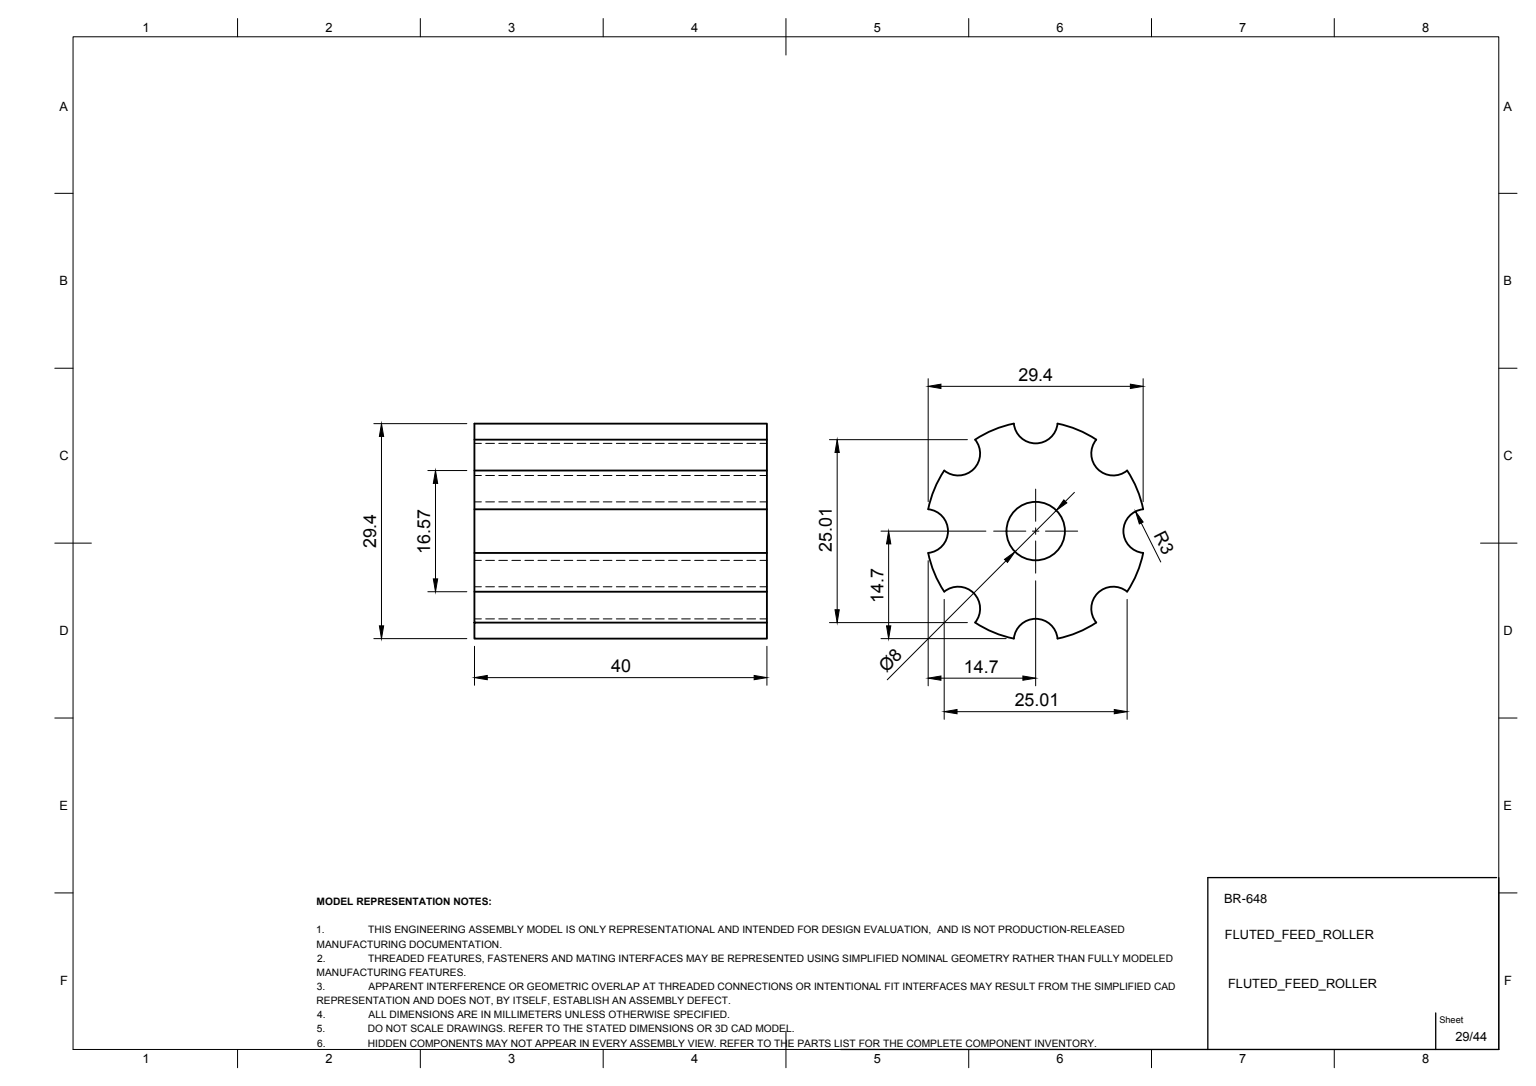
ISO-10303-21;
HEADER;
FILE_DESCRIPTION((''),'2;1');
FILE_NAME('FLUTED_FEED_ROLLER.step','2026-10-01T22:05:39-07:00',(''),(''),'','','');
FILE_SCHEMA (('AUTOMOTIVE_DESIGN { 1 0 10303 214 3 1 1 }'));
ENDSEC;
DATA;
#10=MECHANICAL_DESIGN_GEOMETRIC_PRESENTATION_REPRESENTATION('',(#627),#24628);
#543=SHAPE_REPRESENTATION_RELATIONSHIP('SRR','None',#24816,#585) ;
#585=ADVANCED_BREP_SHAPE_REPRESENTATION('',(#666),#24606) ;
#627=STYLED_ITEM('',(#25036),#666) ;
#666=MANIFOLD_SOLID_BREP('FLUTED_FEED_ROLLER',#13169) ;
#884=FACE_BOUND('',#4472,.T.) ;
#885=FACE_BOUND('',#4488,.T.) ;
#1542=LINE('',#23181,#2378) ;
#1543=LINE('',#23188,#2379) ;
#1544=LINE('',#23191,#2380) ;
#1545=LINE('',#23225,#2381) ;
#1546=LINE('',#23229,#2382) ;
#1547=LINE('',#23233,#2383) ;
#1548=LINE('',#23237,#2384) ;
#1549=LINE('',#23241,#2385) ;
#1550=LINE('',#23245,#2386) ;
#1551=LINE('',#23249,#2387) ;
#1552=LINE('',#23253,#2388) ;
#1553=LINE('',#23257,#2389) ;
#1554=LINE('',#23261,#2390) ;
#1555=LINE('',#23265,#2391) ;
#1556=LINE('',#23269,#2392) ;
#1557=LINE('',#23273,#2393) ;
#1558=LINE('',#23277,#2394) ;
#2378=VECTOR('',#18511,0.4) ;
#2379=VECTOR('',#18518,1.) ;
#2380=VECTOR('',#18521,1.) ;
#2381=VECTOR('',#18558,1.) ;
#2382=VECTOR('',#18563,1.) ;
#2383=VECTOR('',#18568,1.) ;
#2384=VECTOR('',#18573,1.) ;
#2385=VECTOR('',#18578,1.) ;
#2386=VECTOR('',#18583,1.) ;
#2387=VECTOR('',#18588,1.) ;
#2388=VECTOR('',#18593,1.) ;
#2389=VECTOR('',#18598,1.) ;
#2390=VECTOR('',#18603,1.) ;
#2391=VECTOR('',#18608,1.) ;
#2392=VECTOR('',#18613,1.) ;
#2393=VECTOR('',#18618,1.) ;
#2394=VECTOR('',#18623,1.) ;
#2880=CYLINDRICAL_SURFACE('',#14940,0.4) ;
#2881=CYLINDRICAL_SURFACE('',#14943,0.3) ;
#2882=CYLINDRICAL_SURFACE('',#14962,1.5) ;
#2883=CYLINDRICAL_SURFACE('',#14964,0.3) ;
#2884=CYLINDRICAL_SURFACE('',#14966,1.5) ;
#2885=CYLINDRICAL_SURFACE('',#14968,0.3) ;
#2886=CYLINDRICAL_SURFACE('',#14970,1.5) ;
#2887=CYLINDRICAL_SURFACE('',#14972,0.3) ;
#2888=CYLINDRICAL_SURFACE('',#14974,1.5) ;
#2889=CYLINDRICAL_SURFACE('',#14976,0.3) ;
#2890=CYLINDRICAL_SURFACE('',#14978,1.5) ;
#2891=CYLINDRICAL_SURFACE('',#14980,0.3) ;
#2892=CYLINDRICAL_SURFACE('',#14982,1.5) ;
#2893=CYLINDRICAL_SURFACE('',#14984,0.3) ;
#2894=CYLINDRICAL_SURFACE('',#14986,1.5) ;
#2895=CYLINDRICAL_SURFACE('',#14988,0.3) ;
#2896=CYLINDRICAL_SURFACE('',#14992,1.5) ;
#3504=FACE_OUTER_BOUND('',#4469,.T.) ;
#3505=FACE_OUTER_BOUND('',#4470,.T.) ;
#3506=FACE_OUTER_BOUND('',#4471,.T.) ;
#3507=FACE_OUTER_BOUND('',#4473,.T.) ;
#3508=FACE_OUTER_BOUND('',#4474,.T.) ;
#3509=FACE_OUTER_BOUND('',#4475,.T.) ;
#3510=FACE_OUTER_BOUND('',#4476,.T.) ;
#3511=FACE_OUTER_BOUND('',#4477,.T.) ;
#3512=FACE_OUTER_BOUND('',#4478,.T.) ;
#3513=FACE_OUTER_BOUND('',#4479,.T.) ;
#3514=FACE_OUTER_BOUND('',#4480,.T.) ;
#3515=FACE_OUTER_BOUND('',#4481,.T.) ;
#3516=FACE_OUTER_BOUND('',#4482,.T.) ;
#3517=FACE_OUTER_BOUND('',#4483,.T.) ;
#3518=FACE_OUTER_BOUND('',#4484,.T.) ;
#3519=FACE_OUTER_BOUND('',#4485,.T.) ;
#3520=FACE_OUTER_BOUND('',#4486,.T.) ;
#3521=FACE_OUTER_BOUND('',#4487,.T.) ;
#3522=FACE_OUTER_BOUND('',#4489,.T.) ;
#4469=EDGE_LOOP('',(#11027,#11028,#11029,#11030)) ;
#4470=EDGE_LOOP('',(#11031,#11032,#11033,#11034)) ;
#4471=EDGE_LOOP('',(#11035,#11036,#11037,#11038,#11039,#11040,#11041,#11042,
#11043,#11044,#11045,#11046,#11047,#11048,#11049,#11050)) ;
#4472=EDGE_LOOP('',(#11051)) ;
#4473=EDGE_LOOP('',(#11052,#11053,#11054,#11055)) ;
#4474=EDGE_LOOP('',(#11056,#11057,#11058,#11059)) ;
#4475=EDGE_LOOP('',(#11060,#11061,#11062,#11063)) ;
#4476=EDGE_LOOP('',(#11064,#11065,#11066,#11067)) ;
#4477=EDGE_LOOP('',(#11068,#11069,#11070,#11071)) ;
#4478=EDGE_LOOP('',(#11072,#11073,#11074,#11075)) ;
#4479=EDGE_LOOP('',(#11076,#11077,#11078,#11079)) ;
#4480=EDGE_LOOP('',(#11080,#11081,#11082,#11083)) ;
#4481=EDGE_LOOP('',(#11084,#11085,#11086,#11087)) ;
#4482=EDGE_LOOP('',(#11088,#11089,#11090,#11091)) ;
#4483=EDGE_LOOP('',(#11092,#11093,#11094,#11095)) ;
#4484=EDGE_LOOP('',(#11096,#11097,#11098,#11099)) ;
#4485=EDGE_LOOP('',(#11100,#11101,#11102,#11103)) ;
#4486=EDGE_LOOP('',(#11104,#11105,#11106,#11107)) ;
#4487=EDGE_LOOP('',(#11108,#11109,#11110,#11111,#11112,#11113,#11114,#11115,
#11116,#11117,#11118,#11119,#11120,#11121,#11122,#11123)) ;
#4488=EDGE_LOOP('',(#11124)) ;
#4489=EDGE_LOOP('',(#11125,#11126,#11127,#11128)) ;
#5371=CIRCLE('',#14941,0.4) ;
#5372=CIRCLE('',#14942,0.4) ;
#5373=CIRCLE('',#14944,0.3) ;
#5374=CIRCLE('',#14945,0.3) ;
#5375=CIRCLE('',#14947,1.5) ;
#5376=CIRCLE('',#14948,0.3) ;
#5377=CIRCLE('',#14949,1.5) ;
#5378=CIRCLE('',#14950,0.3) ;
#5379=CIRCLE('',#14951,1.5) ;
#5380=CIRCLE('',#14952,0.3) ;
#5381=CIRCLE('',#14953,1.5) ;
#5382=CIRCLE('',#14954,0.3) ;
#5383=CIRCLE('',#14955,1.5) ;
#5384=CIRCLE('',#14956,0.3) ;
#5385=CIRCLE('',#14957,1.5) ;
#5386=CIRCLE('',#14958,0.3) ;
#5387=CIRCLE('',#14959,1.5) ;
#5388=CIRCLE('',#14960,0.3) ;
#5389=CIRCLE('',#14961,1.5) ;
#5390=CIRCLE('',#14963,1.5) ;
#5391=CIRCLE('',#14965,0.3) ;
#5392=CIRCLE('',#14967,1.5) ;
#5393=CIRCLE('',#14969,0.3) ;
#5394=CIRCLE('',#14971,1.5) ;
#5395=CIRCLE('',#14973,0.3) ;
#5396=CIRCLE('',#14975,1.5) ;
#5397=CIRCLE('',#14977,0.3) ;
#5398=CIRCLE('',#14979,1.5) ;
#5399=CIRCLE('',#14981,0.3) ;
#5400=CIRCLE('',#14983,1.5) ;
#5401=CIRCLE('',#14985,0.3) ;
#5402=CIRCLE('',#14987,1.5) ;
#5403=CIRCLE('',#14989,0.3) ;
#5404=CIRCLE('',#14991,1.5) ;
#6413=VERTEX_POINT('',#23178) ;
#6414=VERTEX_POINT('',#23180) ;
#6415=VERTEX_POINT('',#23184) ;
#6416=VERTEX_POINT('',#23185) ;
#6417=VERTEX_POINT('',#23187) ;
#6418=VERTEX_POINT('',#23189) ;
#6419=VERTEX_POINT('',#23193) ;
#6420=VERTEX_POINT('',#23195) ;
#6421=VERTEX_POINT('',#23197) ;
#6422=VERTEX_POINT('',#23199) ;
#6423=VERTEX_POINT('',#23201) ;
#6424=VERTEX_POINT('',#23203) ;
#6425=VERTEX_POINT('',#23205) ;
#6426=VERTEX_POINT('',#23207) ;
#6427=VERTEX_POINT('',#23209) ;
#6428=VERTEX_POINT('',#23211) ;
#6429=VERTEX_POINT('',#23213) ;
#6430=VERTEX_POINT('',#23215) ;
#6431=VERTEX_POINT('',#23217) ;
#6432=VERTEX_POINT('',#23219) ;
#6433=VERTEX_POINT('',#23223) ;
#6434=VERTEX_POINT('',#23227) ;
#6435=VERTEX_POINT('',#23231) ;
#6436=VERTEX_POINT('',#23235) ;
#6437=VERTEX_POINT('',#23239) ;
#6438=VERTEX_POINT('',#23243) ;
#6439=VERTEX_POINT('',#23247) ;
#6440=VERTEX_POINT('',#23251) ;
#6441=VERTEX_POINT('',#23255) ;
#6442=VERTEX_POINT('',#23259) ;
#6443=VERTEX_POINT('',#23263) ;
#6444=VERTEX_POINT('',#23267) ;
#6445=VERTEX_POINT('',#23271) ;
#6446=VERTEX_POINT('',#23275) ;
#8003=EDGE_CURVE('',#6413,#6413,#5371,.T.) ;
#8004=EDGE_CURVE('',#6413,#6414,#1542,.T.) ;
#8005=EDGE_CURVE('',#6414,#6414,#5372,.T.) ;
#8006=EDGE_CURVE('',#6415,#6416,#5373,.T.) ;
#8007=EDGE_CURVE('',#6417,#6415,#1543,.T.) ;
#8008=EDGE_CURVE('',#6418,#6417,#5374,.T.) ;
#8009=EDGE_CURVE('',#6416,#6418,#1544,.T.) ;
#8010=EDGE_CURVE('',#6417,#6419,#5375,.T.) ;
#8011=EDGE_CURVE('',#6419,#6420,#5376,.T.) ;
#8012=EDGE_CURVE('',#6420,#6421,#5377,.T.) ;
#8013=EDGE_CURVE('',#6421,#6422,#5378,.T.) ;
#8014=EDGE_CURVE('',#6422,#6423,#5379,.T.) ;
#8015=EDGE_CURVE('',#6423,#6424,#5380,.T.) ;
#8016=EDGE_CURVE('',#6424,#6425,#5381,.T.) ;
#8017=EDGE_CURVE('',#6425,#6426,#5382,.T.) ;
#8018=EDGE_CURVE('',#6426,#6427,#5383,.T.) ;
#8019=EDGE_CURVE('',#6427,#6428,#5384,.T.) ;
#8020=EDGE_CURVE('',#6428,#6429,#5385,.T.) ;
#8021=EDGE_CURVE('',#6429,#6430,#5386,.T.) ;
#8022=EDGE_CURVE('',#6430,#6431,#5387,.T.) ;
#8023=EDGE_CURVE('',#6431,#6432,#5388,.T.) ;
#8024=EDGE_CURVE('',#6432,#6418,#5389,.T.) ;
#8025=EDGE_CURVE('',#6433,#6415,#5390,.T.) ;
#8026=EDGE_CURVE('',#6433,#6419,#1545,.T.) ;
#8027=EDGE_CURVE('',#6434,#6433,#5391,.T.) ;
#8028=EDGE_CURVE('',#6420,#6434,#1546,.T.) ;
#8029=EDGE_CURVE('',#6435,#6434,#5392,.T.) ;
#8030=EDGE_CURVE('',#6435,#6421,#1547,.T.) ;
#8031=EDGE_CURVE('',#6436,#6435,#5393,.T.) ;
#8032=EDGE_CURVE('',#6422,#6436,#1548,.T.) ;
#8033=EDGE_CURVE('',#6437,#6436,#5394,.T.) ;
#8034=EDGE_CURVE('',#6437,#6423,#1549,.T.) ;
#8035=EDGE_CURVE('',#6438,#6437,#5395,.T.) ;
#8036=EDGE_CURVE('',#6424,#6438,#1550,.T.) ;
#8037=EDGE_CURVE('',#6439,#6438,#5396,.T.) ;
#8038=EDGE_CURVE('',#6439,#6425,#1551,.T.) ;
#8039=EDGE_CURVE('',#6440,#6439,#5397,.T.) ;
#8040=EDGE_CURVE('',#6426,#6440,#1552,.T.) ;
#8041=EDGE_CURVE('',#6441,#6440,#5398,.T.) ;
#8042=EDGE_CURVE('',#6441,#6427,#1553,.T.) ;
#8043=EDGE_CURVE('',#6442,#6441,#5399,.T.) ;
#8044=EDGE_CURVE('',#6428,#6442,#1554,.T.) ;
#8045=EDGE_CURVE('',#6443,#6442,#5400,.T.) ;
#8046=EDGE_CURVE('',#6443,#6429,#1555,.T.) ;
#8047=EDGE_CURVE('',#6444,#6443,#5401,.T.) ;
#8048=EDGE_CURVE('',#6430,#6444,#1556,.T.) ;
#8049=EDGE_CURVE('',#6445,#6444,#5402,.T.) ;
#8050=EDGE_CURVE('',#6445,#6431,#1557,.T.) ;
#8051=EDGE_CURVE('',#6446,#6445,#5403,.T.) ;
#8052=EDGE_CURVE('',#6432,#6446,#1558,.T.) ;
#8053=EDGE_CURVE('',#6416,#6446,#5404,.T.) ;
#11027=ORIENTED_EDGE('',*,*,#8003,.F.) ;
#11028=ORIENTED_EDGE('',*,*,#8004,.T.) ;
#11029=ORIENTED_EDGE('',*,*,#8005,.F.) ;
#11030=ORIENTED_EDGE('',*,*,#8004,.F.) ;
#11031=ORIENTED_EDGE('',*,*,#8006,.F.) ;
#11032=ORIENTED_EDGE('',*,*,#8007,.F.) ;
#11033=ORIENTED_EDGE('',*,*,#8008,.F.) ;
#11034=ORIENTED_EDGE('',*,*,#8009,.F.) ;
#11035=ORIENTED_EDGE('',*,*,#8008,.T.) ;
#11036=ORIENTED_EDGE('',*,*,#8010,.T.) ;
#11037=ORIENTED_EDGE('',*,*,#8011,.T.) ;
#11038=ORIENTED_EDGE('',*,*,#8012,.T.) ;
#11039=ORIENTED_EDGE('',*,*,#8013,.T.) ;
#11040=ORIENTED_EDGE('',*,*,#8014,.T.) ;
#11041=ORIENTED_EDGE('',*,*,#8015,.T.) ;
#11042=ORIENTED_EDGE('',*,*,#8016,.T.) ;
#11043=ORIENTED_EDGE('',*,*,#8017,.T.) ;
#11044=ORIENTED_EDGE('',*,*,#8018,.T.) ;
#11045=ORIENTED_EDGE('',*,*,#8019,.T.) ;
#11046=ORIENTED_EDGE('',*,*,#8020,.T.) ;
#11047=ORIENTED_EDGE('',*,*,#8021,.T.) ;
#11048=ORIENTED_EDGE('',*,*,#8022,.T.) ;
#11049=ORIENTED_EDGE('',*,*,#8023,.T.) ;
#11050=ORIENTED_EDGE('',*,*,#8024,.T.) ;
#11051=ORIENTED_EDGE('',*,*,#8005,.T.) ;
#11052=ORIENTED_EDGE('',*,*,#8007,.T.) ;
#11053=ORIENTED_EDGE('',*,*,#8025,.F.) ;
#11054=ORIENTED_EDGE('',*,*,#8026,.T.) ;
#11055=ORIENTED_EDGE('',*,*,#8010,.F.) ;
#11056=ORIENTED_EDGE('',*,*,#8027,.F.) ;
#11057=ORIENTED_EDGE('',*,*,#8028,.F.) ;
#11058=ORIENTED_EDGE('',*,*,#8011,.F.) ;
#11059=ORIENTED_EDGE('',*,*,#8026,.F.) ;
#11060=ORIENTED_EDGE('',*,*,#8028,.T.) ;
#11061=ORIENTED_EDGE('',*,*,#8029,.F.) ;
#11062=ORIENTED_EDGE('',*,*,#8030,.T.) ;
#11063=ORIENTED_EDGE('',*,*,#8012,.F.) ;
#11064=ORIENTED_EDGE('',*,*,#8031,.F.) ;
#11065=ORIENTED_EDGE('',*,*,#8032,.F.) ;
#11066=ORIENTED_EDGE('',*,*,#8013,.F.) ;
#11067=ORIENTED_EDGE('',*,*,#8030,.F.) ;
#11068=ORIENTED_EDGE('',*,*,#8032,.T.) ;
#11069=ORIENTED_EDGE('',*,*,#8033,.F.) ;
#11070=ORIENTED_EDGE('',*,*,#8034,.T.) ;
#11071=ORIENTED_EDGE('',*,*,#8014,.F.) ;
#11072=ORIENTED_EDGE('',*,*,#8035,.F.) ;
#11073=ORIENTED_EDGE('',*,*,#8036,.F.) ;
#11074=ORIENTED_EDGE('',*,*,#8015,.F.) ;
#11075=ORIENTED_EDGE('',*,*,#8034,.F.) ;
#11076=ORIENTED_EDGE('',*,*,#8036,.T.) ;
#11077=ORIENTED_EDGE('',*,*,#8037,.F.) ;
#11078=ORIENTED_EDGE('',*,*,#8038,.T.) ;
#11079=ORIENTED_EDGE('',*,*,#8016,.F.) ;
#11080=ORIENTED_EDGE('',*,*,#8039,.F.) ;
#11081=ORIENTED_EDGE('',*,*,#8040,.F.) ;
#11082=ORIENTED_EDGE('',*,*,#8017,.F.) ;
#11083=ORIENTED_EDGE('',*,*,#8038,.F.) ;
#11084=ORIENTED_EDGE('',*,*,#8040,.T.) ;
#11085=ORIENTED_EDGE('',*,*,#8041,.F.) ;
#11086=ORIENTED_EDGE('',*,*,#8042,.T.) ;
#11087=ORIENTED_EDGE('',*,*,#8018,.F.) ;
#11088=ORIENTED_EDGE('',*,*,#8043,.F.) ;
#11089=ORIENTED_EDGE('',*,*,#8044,.F.) ;
#11090=ORIENTED_EDGE('',*,*,#8019,.F.) ;
#11091=ORIENTED_EDGE('',*,*,#8042,.F.) ;
#11092=ORIENTED_EDGE('',*,*,#8044,.T.) ;
#11093=ORIENTED_EDGE('',*,*,#8045,.F.) ;
#11094=ORIENTED_EDGE('',*,*,#8046,.T.) ;
#11095=ORIENTED_EDGE('',*,*,#8020,.F.) ;
#11096=ORIENTED_EDGE('',*,*,#8047,.F.) ;
#11097=ORIENTED_EDGE('',*,*,#8048,.F.) ;
#11098=ORIENTED_EDGE('',*,*,#8021,.F.) ;
#11099=ORIENTED_EDGE('',*,*,#8046,.F.) ;
#11100=ORIENTED_EDGE('',*,*,#8048,.T.) ;
#11101=ORIENTED_EDGE('',*,*,#8049,.F.) ;
#11102=ORIENTED_EDGE('',*,*,#8050,.T.) ;
#11103=ORIENTED_EDGE('',*,*,#8022,.F.) ;
#11104=ORIENTED_EDGE('',*,*,#8050,.F.) ;
#11105=ORIENTED_EDGE('',*,*,#8051,.F.) ;
#11106=ORIENTED_EDGE('',*,*,#8052,.F.) ;
#11107=ORIENTED_EDGE('',*,*,#8023,.F.) ;
#11108=ORIENTED_EDGE('',*,*,#8006,.T.) ;
#11109=ORIENTED_EDGE('',*,*,#8053,.T.) ;
#11110=ORIENTED_EDGE('',*,*,#8051,.T.) ;
#11111=ORIENTED_EDGE('',*,*,#8049,.T.) ;
#11112=ORIENTED_EDGE('',*,*,#8047,.T.) ;
#11113=ORIENTED_EDGE('',*,*,#8045,.T.) ;
#11114=ORIENTED_EDGE('',*,*,#8043,.T.) ;
#11115=ORIENTED_EDGE('',*,*,#8041,.T.) ;
#11116=ORIENTED_EDGE('',*,*,#8039,.T.) ;
#11117=ORIENTED_EDGE('',*,*,#8037,.T.) ;
#11118=ORIENTED_EDGE('',*,*,#8035,.T.) ;
#11119=ORIENTED_EDGE('',*,*,#8033,.T.) ;
#11120=ORIENTED_EDGE('',*,*,#8031,.T.) ;
#11121=ORIENTED_EDGE('',*,*,#8029,.T.) ;
#11122=ORIENTED_EDGE('',*,*,#8027,.T.) ;
#11123=ORIENTED_EDGE('',*,*,#8025,.T.) ;
#11124=ORIENTED_EDGE('',*,*,#8003,.T.) ;
#11125=ORIENTED_EDGE('',*,*,#8009,.T.) ;
#11126=ORIENTED_EDGE('',*,*,#8024,.F.) ;
#11127=ORIENTED_EDGE('',*,*,#8052,.T.) ;
#11128=ORIENTED_EDGE('',*,*,#8053,.F.) ;
#12209=PLANE('',#14946) ;
#12210=PLANE('',#14990) ;
#12899=ADVANCED_FACE('',(#3504),#2880,.F.) ;
#12900=ADVANCED_FACE('',(#3505),#2881,.F.) ;
#12901=ADVANCED_FACE('',(#3506,#884),#12209,.T.) ;
#12902=ADVANCED_FACE('',(#3507),#2882,.T.) ;
#12903=ADVANCED_FACE('',(#3508),#2883,.F.) ;
#12904=ADVANCED_FACE('',(#3509),#2884,.T.) ;
#12905=ADVANCED_FACE('',(#3510),#2885,.F.) ;
#12906=ADVANCED_FACE('',(#3511),#2886,.T.) ;
#12907=ADVANCED_FACE('',(#3512),#2887,.F.) ;
#12908=ADVANCED_FACE('',(#3513),#2888,.T.) ;
#12909=ADVANCED_FACE('',(#3514),#2889,.F.) ;
#12910=ADVANCED_FACE('',(#3515),#2890,.T.) ;
#12911=ADVANCED_FACE('',(#3516),#2891,.F.) ;
#12912=ADVANCED_FACE('',(#3517),#2892,.T.) ;
#12913=ADVANCED_FACE('',(#3518),#2893,.F.) ;
#12914=ADVANCED_FACE('',(#3519),#2894,.T.) ;
#12915=ADVANCED_FACE('',(#3520),#2895,.F.) ;
#12916=ADVANCED_FACE('',(#3521,#885),#12210,.T.) ;
#12917=ADVANCED_FACE('',(#3522),#2896,.T.) ;
#13169=CLOSED_SHELL('',(#12899,#12900,#12901,#12902,#12903,#12904,#12905,
#12906,#12907,#12908,#12909,#12910,#12911,#12912,#12913,#12914,#12915,#12916,
#12917)) ;
#14939=AXIS2_PLACEMENT_3D('',#23176,#18505,#18506) ;
#14940=AXIS2_PLACEMENT_3D('',#23177,#18507,#18508) ;
#14941=AXIS2_PLACEMENT_3D('',#23179,#18509,#18510) ;
#14942=AXIS2_PLACEMENT_3D('',#23182,#18512,#18513) ;
#14943=AXIS2_PLACEMENT_3D('',#23183,#18514,#18515) ;
#14944=AXIS2_PLACEMENT_3D('',#23186,#18516,#18517) ;
#14945=AXIS2_PLACEMENT_3D('',#23190,#18519,#18520) ;
#14946=AXIS2_PLACEMENT_3D('',#23192,#18522,#18523) ;
#14947=AXIS2_PLACEMENT_3D('',#23194,#18524,#18525) ;
#14948=AXIS2_PLACEMENT_3D('',#23196,#18526,#18527) ;
#14949=AXIS2_PLACEMENT_3D('',#23198,#18528,#18529) ;
#14950=AXIS2_PLACEMENT_3D('',#23200,#18530,#18531) ;
#14951=AXIS2_PLACEMENT_3D('',#23202,#18532,#18533) ;
#14952=AXIS2_PLACEMENT_3D('',#23204,#18534,#18535) ;
#14953=AXIS2_PLACEMENT_3D('',#23206,#18536,#18537) ;
#14954=AXIS2_PLACEMENT_3D('',#23208,#18538,#18539) ;
#14955=AXIS2_PLACEMENT_3D('',#23210,#18540,#18541) ;
#14956=AXIS2_PLACEMENT_3D('',#23212,#18542,#18543) ;
#14957=AXIS2_PLACEMENT_3D('',#23214,#18544,#18545) ;
#14958=AXIS2_PLACEMENT_3D('',#23216,#18546,#18547) ;
#14959=AXIS2_PLACEMENT_3D('',#23218,#18548,#18549) ;
#14960=AXIS2_PLACEMENT_3D('',#23220,#18550,#18551) ;
#14961=AXIS2_PLACEMENT_3D('',#23221,#18552,#18553) ;
#14962=AXIS2_PLACEMENT_3D('',#23222,#18554,#18555) ;
#14963=AXIS2_PLACEMENT_3D('',#23224,#18556,#18557) ;
#14964=AXIS2_PLACEMENT_3D('',#23226,#18559,#18560) ;
#14965=AXIS2_PLACEMENT_3D('',#23228,#18561,#18562) ;
#14966=AXIS2_PLACEMENT_3D('',#23230,#18564,#18565) ;
#14967=AXIS2_PLACEMENT_3D('',#23232,#18566,#18567) ;
#14968=AXIS2_PLACEMENT_3D('',#23234,#18569,#18570) ;
#14969=AXIS2_PLACEMENT_3D('',#23236,#18571,#18572) ;
#14970=AXIS2_PLACEMENT_3D('',#23238,#18574,#18575) ;
#14971=AXIS2_PLACEMENT_3D('',#23240,#18576,#18577) ;
#14972=AXIS2_PLACEMENT_3D('',#23242,#18579,#18580) ;
#14973=AXIS2_PLACEMENT_3D('',#23244,#18581,#18582) ;
#14974=AXIS2_PLACEMENT_3D('',#23246,#18584,#18585) ;
#14975=AXIS2_PLACEMENT_3D('',#23248,#18586,#18587) ;
#14976=AXIS2_PLACEMENT_3D('',#23250,#18589,#18590) ;
#14977=AXIS2_PLACEMENT_3D('',#23252,#18591,#18592) ;
#14978=AXIS2_PLACEMENT_3D('',#23254,#18594,#18595) ;
#14979=AXIS2_PLACEMENT_3D('',#23256,#18596,#18597) ;
#14980=AXIS2_PLACEMENT_3D('',#23258,#18599,#18600) ;
#14981=AXIS2_PLACEMENT_3D('',#23260,#18601,#18602) ;
#14982=AXIS2_PLACEMENT_3D('',#23262,#18604,#18605) ;
#14983=AXIS2_PLACEMENT_3D('',#23264,#18606,#18607) ;
#14984=AXIS2_PLACEMENT_3D('',#23266,#18609,#18610) ;
#14985=AXIS2_PLACEMENT_3D('',#23268,#18611,#18612) ;
#14986=AXIS2_PLACEMENT_3D('',#23270,#18614,#18615) ;
#14987=AXIS2_PLACEMENT_3D('',#23272,#18616,#18617) ;
#14988=AXIS2_PLACEMENT_3D('',#23274,#18619,#18620) ;
#14989=AXIS2_PLACEMENT_3D('',#23276,#18621,#18622) ;
#14990=AXIS2_PLACEMENT_3D('',#23278,#18624,#18625) ;
#14991=AXIS2_PLACEMENT_3D('',#23279,#18626,#18627) ;
#14992=AXIS2_PLACEMENT_3D('',#23280,#18628,#18629) ;
#18505=DIRECTION('axis',(0.,0.,1.)) ;
#18506=DIRECTION('refdir',(1.,0.,0.)) ;
#18507=DIRECTION('center_axis',(0.,1.,0.)) ;
#18508=DIRECTION('ref_axis',(1.,0.,0.)) ;
#18509=DIRECTION('center_axis',(0.,1.,0.)) ;
#18510=DIRECTION('ref_axis',(1.,0.,0.)) ;
#18511=DIRECTION('',(0.,1.,0.)) ;
#18512=DIRECTION('center_axis',(0.,-1.,0.)) ;
#18513=DIRECTION('ref_axis',(1.,0.,0.)) ;
#18514=DIRECTION('center_axis',(0.,1.,0.)) ;
#18515=DIRECTION('ref_axis',(-0.707106781186545,0.,0.70710678118655)) ;
#18516=DIRECTION('center_axis',(0.,1.,0.)) ;
#18517=DIRECTION('ref_axis',(1.,0.,0.)) ;
#18518=DIRECTION('',(0.,-1.,0.)) ;
#18519=DIRECTION('center_axis',(0.,-1.,0.)) ;
#18520=DIRECTION('ref_axis',(1.,0.,0.)) ;
#18521=DIRECTION('',(0.,1.,0.)) ;
#18522=DIRECTION('center_axis',(0.,1.,0.)) ;
#18523=DIRECTION('ref_axis',(1.,0.,0.)) ;
#18524=DIRECTION('center_axis',(0.,1.,0.)) ;
#18525=DIRECTION('ref_axis',(1.,0.,0.)) ;
#18526=DIRECTION('center_axis',(0.,-1.,0.)) ;
#18527=DIRECTION('ref_axis',(1.,0.,0.)) ;
#18528=DIRECTION('center_axis',(0.,1.,0.)) ;
#18529=DIRECTION('ref_axis',(1.,0.,0.)) ;
#18530=DIRECTION('center_axis',(0.,-1.,0.)) ;
#18531=DIRECTION('ref_axis',(1.,0.,0.)) ;
#18532=DIRECTION('center_axis',(0.,1.,0.)) ;
#18533=DIRECTION('ref_axis',(1.,0.,0.)) ;
#18534=DIRECTION('center_axis',(0.,-1.,0.)) ;
#18535=DIRECTION('ref_axis',(1.,0.,0.)) ;
#18536=DIRECTION('center_axis',(0.,1.,0.)) ;
#18537=DIRECTION('ref_axis',(1.,0.,0.)) ;
#18538=DIRECTION('center_axis',(0.,-1.,0.)) ;
#18539=DIRECTION('ref_axis',(1.,0.,0.)) ;
#18540=DIRECTION('center_axis',(0.,1.,0.)) ;
#18541=DIRECTION('ref_axis',(1.,0.,0.)) ;
#18542=DIRECTION('center_axis',(0.,-1.,0.)) ;
#18543=DIRECTION('ref_axis',(1.,0.,0.)) ;
#18544=DIRECTION('center_axis',(0.,1.,0.)) ;
#18545=DIRECTION('ref_axis',(1.,0.,0.)) ;
#18546=DIRECTION('center_axis',(0.,-1.,0.)) ;
#18547=DIRECTION('ref_axis',(1.,0.,0.)) ;
#18548=DIRECTION('center_axis',(0.,1.,0.)) ;
#18549=DIRECTION('ref_axis',(1.,0.,0.)) ;
#18550=DIRECTION('center_axis',(0.,-1.,0.)) ;
#18551=DIRECTION('ref_axis',(1.,0.,0.)) ;
#18552=DIRECTION('center_axis',(0.,1.,0.)) ;
#18553=DIRECTION('ref_axis',(1.,0.,0.)) ;
#18554=DIRECTION('center_axis',(0.,1.,0.)) ;
#18555=DIRECTION('ref_axis',(1.,0.,0.)) ;
#18556=DIRECTION('center_axis',(0.,-1.,0.)) ;
#18557=DIRECTION('ref_axis',(1.,0.,0.)) ;
#18558=DIRECTION('',(0.,1.,0.)) ;
#18559=DIRECTION('center_axis',(0.,1.,0.)) ;
#18560=DIRECTION('ref_axis',(1.,0.,0.)) ;
#18561=DIRECTION('center_axis',(0.,1.,0.)) ;
#18562=DIRECTION('ref_axis',(1.,0.,0.)) ;
#18563=DIRECTION('',(0.,-1.,0.)) ;
#18564=DIRECTION('center_axis',(0.,1.,0.)) ;
#18565=DIRECTION('ref_axis',(1.,0.,0.)) ;
#18566=DIRECTION('center_axis',(0.,-1.,0.)) ;
#18567=DIRECTION('ref_axis',(1.,0.,0.)) ;
#18568=DIRECTION('',(0.,1.,0.)) ;
#18569=DIRECTION('center_axis',(0.,1.,0.)) ;
#18570=DIRECTION('ref_axis',(1.,0.,0.)) ;
#18571=DIRECTION('center_axis',(0.,1.,0.)) ;
#18572=DIRECTION('ref_axis',(1.,0.,0.)) ;
#18573=DIRECTION('',(0.,-1.,0.)) ;
#18574=DIRECTION('center_axis',(0.,1.,0.)) ;
#18575=DIRECTION('ref_axis',(1.,0.,0.)) ;
#18576=DIRECTION('center_axis',(0.,-1.,0.)) ;
#18577=DIRECTION('ref_axis',(1.,0.,0.)) ;
#18578=DIRECTION('',(0.,1.,0.)) ;
#18579=DIRECTION('center_axis',(0.,1.,0.)) ;
#18580=DIRECTION('ref_axis',(1.,0.,0.)) ;
#18581=DIRECTION('center_axis',(0.,1.,0.)) ;
#18582=DIRECTION('ref_axis',(1.,0.,0.)) ;
#18583=DIRECTION('',(0.,-1.,0.)) ;
#18584=DIRECTION('center_axis',(0.,1.,0.)) ;
#18585=DIRECTION('ref_axis',(1.,0.,0.)) ;
#18586=DIRECTION('center_axis',(0.,-1.,0.)) ;
#18587=DIRECTION('ref_axis',(1.,0.,0.)) ;
#18588=DIRECTION('',(0.,1.,0.)) ;
#18589=DIRECTION('center_axis',(0.,1.,0.)) ;
#18590=DIRECTION('ref_axis',(1.,0.,0.)) ;
#18591=DIRECTION('center_axis',(0.,1.,0.)) ;
#18592=DIRECTION('ref_axis',(1.,0.,0.)) ;
#18593=DIRECTION('',(0.,-1.,0.)) ;
#18594=DIRECTION('center_axis',(0.,1.,0.)) ;
#18595=DIRECTION('ref_axis',(1.,0.,0.)) ;
#18596=DIRECTION('center_axis',(0.,-1.,0.)) ;
#18597=DIRECTION('ref_axis',(1.,0.,0.)) ;
#18598=DIRECTION('',(0.,1.,0.)) ;
#18599=DIRECTION('center_axis',(0.,1.,0.)) ;
#18600=DIRECTION('ref_axis',(1.,0.,0.)) ;
#18601=DIRECTION('center_axis',(0.,1.,0.)) ;
#18602=DIRECTION('ref_axis',(1.,0.,0.)) ;
#18603=DIRECTION('',(0.,-1.,0.)) ;
#18604=DIRECTION('center_axis',(0.,1.,0.)) ;
#18605=DIRECTION('ref_axis',(1.,0.,0.)) ;
#18606=DIRECTION('center_axis',(0.,-1.,0.)) ;
#18607=DIRECTION('ref_axis',(1.,0.,0.)) ;
#18608=DIRECTION('',(0.,1.,0.)) ;
#18609=DIRECTION('center_axis',(0.,1.,0.)) ;
#18610=DIRECTION('ref_axis',(-0.707106781186545,0.,-0.70710678118655)) ;
#18611=DIRECTION('center_axis',(0.,1.,0.)) ;
#18612=DIRECTION('ref_axis',(1.,0.,0.)) ;
#18613=DIRECTION('',(0.,-1.,0.)) ;
#18614=DIRECTION('center_axis',(0.,1.,0.)) ;
#18615=DIRECTION('ref_axis',(1.,0.,0.)) ;
#18616=DIRECTION('center_axis',(0.,-1.,0.)) ;
#18617=DIRECTION('ref_axis',(1.,0.,0.)) ;
#18618=DIRECTION('',(0.,1.,0.)) ;
#18619=DIRECTION('center_axis',(0.,1.,0.)) ;
#18620=DIRECTION('ref_axis',(-1.,0.,1.22464679914735E-16)) ;
#18621=DIRECTION('center_axis',(0.,1.,0.)) ;
#18622=DIRECTION('ref_axis',(1.,0.,0.)) ;
#18623=DIRECTION('',(0.,-1.,0.)) ;
#18624=DIRECTION('center_axis',(0.,-1.,0.)) ;
#18625=DIRECTION('ref_axis',(-1.,0.,0.)) ;
#18626=DIRECTION('center_axis',(0.,-1.,0.)) ;
#18627=DIRECTION('ref_axis',(1.,0.,0.)) ;
#18628=DIRECTION('center_axis',(0.,1.,0.)) ;
#18629=DIRECTION('ref_axis',(1.,0.,0.)) ;
#23176=CARTESIAN_POINT('',(0.,0.,0.)) ;
#23177=CARTESIAN_POINT('Origin',(-23.,-1.8,-2.2)) ;
#23178=CARTESIAN_POINT('',(-23.4,-3.8,-2.2)) ;
#23179=CARTESIAN_POINT('Origin',(-23.,-3.8,-2.2)) ;
#23180=CARTESIAN_POINT('',(-23.4,0.2,-2.2)) ;
#23181=CARTESIAN_POINT('',(-23.4,-1.8,-2.2)) ;
#23182=CARTESIAN_POINT('Origin',(-23.,0.2,-2.2)) ;
#23183=CARTESIAN_POINT('Origin',(-21.9393398282202,-1.8,-3.26066017177982)) ;
#23184=CARTESIAN_POINT('',(-22.1716217408478,-3.8,-3.45051567753628)) ;
#23185=CARTESIAN_POINT('',(-21.7494843224637,-3.8,-3.02837825915217)) ;
#23186=CARTESIAN_POINT('Origin',(-21.9393398282202,-3.8,-3.26066017177982)) ;
#23187=CARTESIAN_POINT('',(-22.1716217408478,0.2,-3.45051567753628)) ;
#23188=CARTESIAN_POINT('',(-22.1716217408478,-1.8,-3.45051567753628)) ;
#23189=CARTESIAN_POINT('',(-21.7494843224637,0.2,-3.02837825915217)) ;
#23190=CARTESIAN_POINT('Origin',(-21.9393398282202,0.2,-3.26066017177982)) ;
#23191=CARTESIAN_POINT('',(-21.7494843224637,-1.8,-3.02837825915217)) ;
#23192=CARTESIAN_POINT('Origin',(-23.,0.2,-2.2)) ;
#23193=CARTESIAN_POINT('',(-22.701503768868,0.2,-3.67)) ;
#23194=CARTESIAN_POINT('Origin',(-23.,0.2,-2.2)) ;
#23195=CARTESIAN_POINT('',(-23.298496231132,0.2,-3.67)) ;
#23196=CARTESIAN_POINT('Origin',(-23.,0.2,-3.7)) ;
#23197=CARTESIAN_POINT('',(-23.8283782591522,0.2,-3.45051567753628)) ;
#23198=CARTESIAN_POINT('Origin',(-23.,0.2,-2.2)) ;
#23199=CARTESIAN_POINT('',(-24.2505156775363,0.2,-3.02837825915217)) ;
#23200=CARTESIAN_POINT('Origin',(-24.0606601717798,0.2,-3.26066017177982)) ;
#23201=CARTESIAN_POINT('',(-24.47,0.2,-2.49849623113198)) ;
#23202=CARTESIAN_POINT('Origin',(-23.,0.2,-2.2)) ;
#23203=CARTESIAN_POINT('',(-24.47,0.2,-1.90150376886801)) ;
#23204=CARTESIAN_POINT('Origin',(-24.5,0.2,-2.2)) ;
#23205=CARTESIAN_POINT('',(-24.2505156775363,0.2,-1.37162174084783)) ;
#23206=CARTESIAN_POINT('Origin',(-23.,0.2,-2.2)) ;
#23207=CARTESIAN_POINT('',(-23.8283782591522,0.2,-0.949484322463722)) ;
#23208=CARTESIAN_POINT('Origin',(-24.0606601717798,0.2,-1.13933982822018)) ;
#23209=CARTESIAN_POINT('',(-23.298496231132,0.2,-0.73)) ;
#23210=CARTESIAN_POINT('Origin',(-23.,0.2,-2.2)) ;
#23211=CARTESIAN_POINT('',(-22.701503768868,0.2,-0.73)) ;
#23212=CARTESIAN_POINT('Origin',(-23.,0.2,-0.7)) ;
#23213=CARTESIAN_POINT('',(-22.1716217408478,0.2,-0.94948432246372)) ;
#23214=CARTESIAN_POINT('Origin',(-23.,0.2,-2.2)) ;
#23215=CARTESIAN_POINT('',(-21.7494843224637,0.2,-1.37162174084783)) ;
#23216=CARTESIAN_POINT('Origin',(-21.9393398282202,0.2,-1.13933982822018)) ;
#23217=CARTESIAN_POINT('',(-21.53,0.2,-1.90150376886802)) ;
#23218=CARTESIAN_POINT('Origin',(-23.,0.2,-2.2)) ;
#23219=CARTESIAN_POINT('',(-21.53,0.2,-2.49849623113198)) ;
#23220=CARTESIAN_POINT('Origin',(-21.5,0.2,-2.2)) ;
#23221=CARTESIAN_POINT('Origin',(-23.,0.2,-2.2)) ;
#23222=CARTESIAN_POINT('Origin',(-23.,-1.8,-2.2)) ;
#23223=CARTESIAN_POINT('',(-22.701503768868,-3.8,-3.67)) ;
#23224=CARTESIAN_POINT('Origin',(-23.,-3.8,-2.2)) ;
#23225=CARTESIAN_POINT('',(-22.701503768868,-1.8,-3.67)) ;
#23226=CARTESIAN_POINT('Origin',(-23.,-1.8,-3.7)) ;
#23227=CARTESIAN_POINT('',(-23.298496231132,-3.8,-3.67)) ;
#23228=CARTESIAN_POINT('Origin',(-23.,-3.8,-3.7)) ;
#23229=CARTESIAN_POINT('',(-23.298496231132,-1.8,-3.67)) ;
#23230=CARTESIAN_POINT('Origin',(-23.,-1.8,-2.2)) ;
#23231=CARTESIAN_POINT('',(-23.8283782591522,-3.8,-3.45051567753628)) ;
#23232=CARTESIAN_POINT('Origin',(-23.,-3.8,-2.2)) ;
#23233=CARTESIAN_POINT('',(-23.8283782591522,-1.8,-3.45051567753628)) ;
#23234=CARTESIAN_POINT('Origin',(-24.0606601717798,-1.8,-3.26066017177982)) ;
#23235=CARTESIAN_POINT('',(-24.2505156775363,-3.8,-3.02837825915217)) ;
#23236=CARTESIAN_POINT('Origin',(-24.0606601717798,-3.8,-3.26066017177982)) ;
#23237=CARTESIAN_POINT('',(-24.2505156775363,-1.8,-3.02837825915217)) ;
#23238=CARTESIAN_POINT('Origin',(-23.,-1.8,-2.2)) ;
#23239=CARTESIAN_POINT('',(-24.47,-3.8,-2.49849623113198)) ;
#23240=CARTESIAN_POINT('Origin',(-23.,-3.8,-2.2)) ;
#23241=CARTESIAN_POINT('',(-24.47,-1.8,-2.49849623113199)) ;
#23242=CARTESIAN_POINT('Origin',(-24.5,-1.8,-2.2)) ;
#23243=CARTESIAN_POINT('',(-24.47,-3.8,-1.90150376886801)) ;
#23244=CARTESIAN_POINT('Origin',(-24.5,-3.8,-2.2)) ;
#23245=CARTESIAN_POINT('',(-24.47,-1.8,-1.90150376886801)) ;
#23246=CARTESIAN_POINT('Origin',(-23.,-1.8,-2.2)) ;
#23247=CARTESIAN_POINT('',(-24.2505156775363,-3.8,-1.37162174084783)) ;
#23248=CARTESIAN_POINT('Origin',(-23.,-3.8,-2.2)) ;
#23249=CARTESIAN_POINT('',(-24.2505156775363,-1.8,-1.37162174084783)) ;
#23250=CARTESIAN_POINT('Origin',(-24.0606601717798,-1.8,-1.13933982822018)) ;
#23251=CARTESIAN_POINT('',(-23.8283782591522,-3.8,-0.949484322463722)) ;
#23252=CARTESIAN_POINT('Origin',(-24.0606601717798,-3.8,-1.13933982822018)) ;
#23253=CARTESIAN_POINT('',(-23.8283782591522,-1.8,-0.949484322463721)) ;
#23254=CARTESIAN_POINT('Origin',(-23.,-1.8,-2.2)) ;
#23255=CARTESIAN_POINT('',(-23.298496231132,-3.8,-0.73)) ;
#23256=CARTESIAN_POINT('Origin',(-23.,-3.8,-2.2)) ;
#23257=CARTESIAN_POINT('',(-23.298496231132,-1.8,-0.73)) ;
#23258=CARTESIAN_POINT('Origin',(-23.,-1.8,-0.7)) ;
#23259=CARTESIAN_POINT('',(-22.701503768868,-3.8,-0.73)) ;
#23260=CARTESIAN_POINT('Origin',(-23.,-3.8,-0.7)) ;
#23261=CARTESIAN_POINT('',(-22.701503768868,-1.8,-0.73)) ;
#23262=CARTESIAN_POINT('Origin',(-23.,-1.8,-2.2)) ;
#23263=CARTESIAN_POINT('',(-22.1716217408478,-3.8,-0.94948432246372)) ;
#23264=CARTESIAN_POINT('Origin',(-23.,-3.8,-2.2)) ;
#23265=CARTESIAN_POINT('',(-22.1716217408478,-1.8,-0.94948432246372)) ;
#23266=CARTESIAN_POINT('Origin',(-21.9393398282202,-1.8,-1.13933982822018)) ;
#23267=CARTESIAN_POINT('',(-21.7494843224637,-3.8,-1.37162174084783)) ;
#23268=CARTESIAN_POINT('Origin',(-21.9393398282202,-3.8,-1.13933982822018)) ;
#23269=CARTESIAN_POINT('',(-21.7494843224637,-1.8,-1.37162174084783)) ;
#23270=CARTESIAN_POINT('Origin',(-23.,-1.8,-2.2)) ;
#23271=CARTESIAN_POINT('',(-21.53,-3.8,-1.90150376886802)) ;
#23272=CARTESIAN_POINT('Origin',(-23.,-3.8,-2.2)) ;
#23273=CARTESIAN_POINT('',(-21.53,-1.8,-1.90150376886801)) ;
#23274=CARTESIAN_POINT('Origin',(-21.5,-1.8,-2.2)) ;
#23275=CARTESIAN_POINT('',(-21.53,-3.8,-2.49849623113198)) ;
#23276=CARTESIAN_POINT('Origin',(-21.5,-3.8,-2.2)) ;
#23277=CARTESIAN_POINT('',(-21.53,-1.8,-2.49849623113199)) ;
#23278=CARTESIAN_POINT('Origin',(-23.,-3.8,-2.2)) ;
#23279=CARTESIAN_POINT('Origin',(-23.,-3.8,-2.2)) ;
#23280=CARTESIAN_POINT('Origin',(-23.,-1.8,-2.2)) ;
#24558=UNCERTAINTY_MEASURE_WITH_UNIT(LENGTH_MEASURE(0.001),#24629,
'DISTANCE_ACCURACY_VALUE',
'Maximum model space distance between geometric entities at asserted c
onnectivities') ;
#24580=UNCERTAINTY_MEASURE_WITH_UNIT(LENGTH_MEASURE(0.001),#24629,
'DISTANCE_ACCURACY_VALUE',
'Maximum model space distance between geometric entities at asserted c
onnectivities') ;
#24606=(
GEOMETRIC_REPRESENTATION_CONTEXT(3)
GLOBAL_UNCERTAINTY_ASSIGNED_CONTEXT((#24558))
GLOBAL_UNIT_ASSIGNED_CONTEXT((#24629,#24631,#24632))
REPRESENTATION_CONTEXT('','3D')
) ;
#24628=(
GEOMETRIC_REPRESENTATION_CONTEXT(3)
GLOBAL_UNCERTAINTY_ASSIGNED_CONTEXT((#24580))
GLOBAL_UNIT_ASSIGNED_CONTEXT((#24629,#24631,#24632))
REPRESENTATION_CONTEXT('','3D')
) ;
#24629=(
LENGTH_UNIT()
NAMED_UNIT(*)
SI_UNIT(.CENTI.,.METRE.)
) ;
#24631=(
NAMED_UNIT(*)
PLANE_ANGLE_UNIT()
SI_UNIT($,.RADIAN.)
) ;
#24632=(
NAMED_UNIT(*)
SI_UNIT($,.STERADIAN.)
SOLID_ANGLE_UNIT()
) ;
#24658=SHAPE_DEFINITION_REPRESENTATION(#24727,#24816) ;
#24727=PRODUCT_DEFINITION_SHAPE('',$,#24864) ;
#24816=SHAPE_REPRESENTATION('',(#14939),#24606) ;
#24838=PRODUCT_DEFINITION_CONTEXT('part definition',#24981,'design') ;
#24864=PRODUCT_DEFINITION('FLUTED_FEED_ROLLER',
'FLUTED_FEED_ROLLER',#24911,#24838) ;
#24911=PRODUCT_DEFINITION_FORMATION('',$,#25008) ;
#24981=APPLICATION_CONTEXT(
'Core Data for Automotive Mechanical Design Process') ;
#24982=PRODUCT_CONTEXT('part definition',#24981,'mechanical') ;
#25008=PRODUCT('FLUTED_FEED_ROLLER','FLUTED_FEED_ROLLER',$,(#24982)) ;
#25036=PRESENTATION_STYLE_ASSIGNMENT((#25046)) ;
#25046=SURFACE_STYLE_USAGE(.BOTH.,#25056) ;
#25056=SURFACE_SIDE_STYLE('',(#25066)) ;
#25066=SURFACE_STYLE_FILL_AREA(#25076) ;
#25076=FILL_AREA_STYLE('Nylon 6-6 (White)',(#25086)) ;
#25086=FILL_AREA_STYLE_COLOUR('Nylon 6-6 (White)',#25096) ;
#25096=COLOUR_RGB('Nylon 6-6 (White)', 0.31764706, 0.68627451, 0.89019608) ;
ENDSEC;
END-ISO-10303-21;
